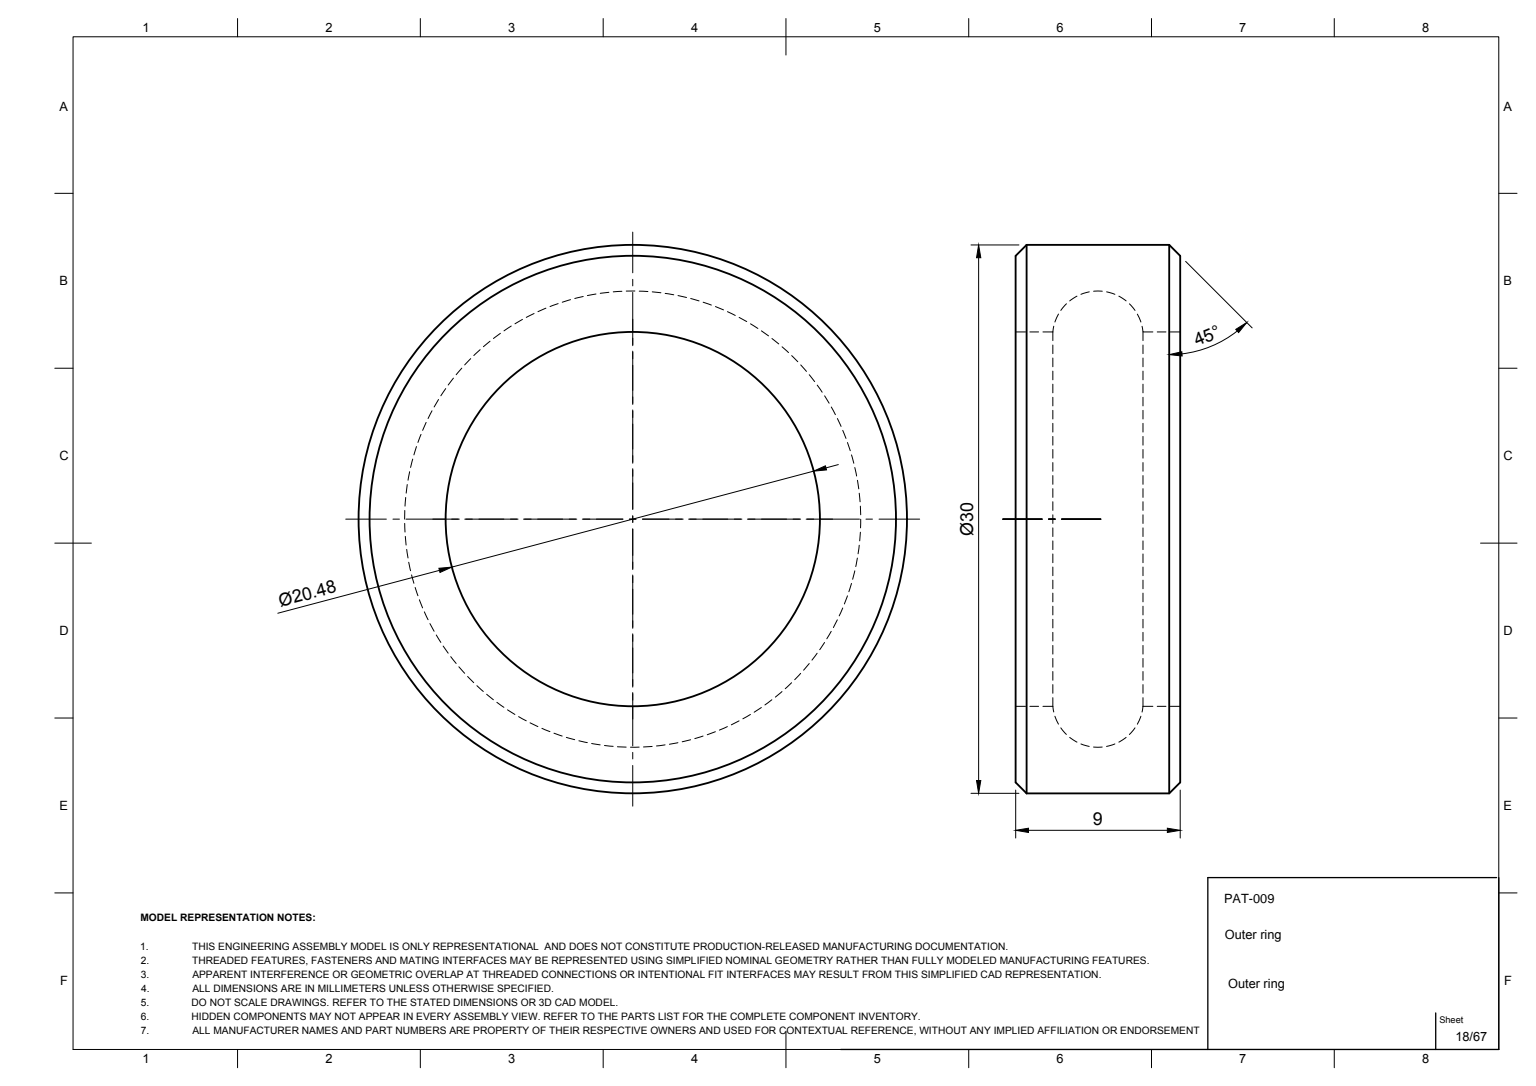
ISO-10303-21;
HEADER;
/* Generated by software containing ST-Developer
 * from STEP Tools, Inc. (www.steptools.com) 
 */

FILE_DESCRIPTION(
/* description */ ('Bell-crank linkage with push rods'),
/* implementation_level */ '2;1');

FILE_NAME(
/* name */ 'Outer ring.step',
/* time_stamp */ '2026-10-28T03:25:15-07:00',
/* author */ (''),
/* organization */ (''),
/* preprocessor_version */ 'ST-DEVELOPER v20.2',
/* originating_system */ 'Autodesk Translation Framework v15.17.0.0',
/* authorisation */ '');

FILE_SCHEMA (('AUTOMOTIVE_DESIGN { 1 0 10303 214 3 1 1 }'));
ENDSEC;

DATA;
#10=MECHANICAL_DESIGN_GEOMETRIC_PRESENTATION_REPRESENTATION('',(#615),#16678);
#432=TOROIDAL_SURFACE('',#9810,1.,0.247676);
#438=CONICAL_SURFACE('',#9821,1.47,0.785398163397449);
#439=CONICAL_SURFACE('',#9825,1.47,0.785398163397449);
#507=SHAPE_REPRESENTATION_RELATIONSHIP('SRR','None',#16924,#561);
#561=ADVANCED_BREP_SHAPE_REPRESENTATION('',(#676),#16629);
#615=STYLED_ITEM('',(#17291),#676);
#676=MANIFOLD_SOLID_BREP('Body1',#8806);
#815=FACE_BOUND('',#2033,.T.);
#816=FACE_BOUND('',#2038,.T.);
#1056=PLANE('',#9818);
#1057=PLANE('',#9827);
#1418=FACE_OUTER_BOUND('',#2030,.T.);
#1419=FACE_OUTER_BOUND('',#2031,.T.);
#1420=FACE_OUTER_BOUND('',#2032,.T.);
#1421=FACE_OUTER_BOUND('',#2034,.T.);
#1422=FACE_OUTER_BOUND('',#2035,.T.);
#1423=FACE_OUTER_BOUND('',#2036,.T.);
#1424=FACE_OUTER_BOUND('',#2037,.T.);
#1425=FACE_OUTER_BOUND('',#2039,.T.);
#2030=EDGE_LOOP('',(#6707,#6708,#6709,#6710,#6711,#6712));
#2031=EDGE_LOOP('',(#6713,#6714,#6715,#6716,#6717));
#2032=EDGE_LOOP('',(#6718));
#2033=EDGE_LOOP('',(#6719));
#2034=EDGE_LOOP('',(#6720,#6721,#6722,#6723));
#2035=EDGE_LOOP('',(#6724,#6725,#6726,#6727));
#2036=EDGE_LOOP('',(#6728,#6729,#6730,#6731));
#2037=EDGE_LOOP('',(#6732));
#2038=EDGE_LOOP('',(#6733));
#2039=EDGE_LOOP('',(#6734,#6735,#6736,#6737,#6738));
#2744=LINE('',#14525,#3293);
#2745=LINE('',#14534,#3294);
#2746=LINE('',#14538,#3295);
#2747=LINE('',#14542,#3296);
#2748=LINE('',#14545,#3297);
#3293=VECTOR('',#11570,1.023815);
#3294=VECTOR('',#11581,1.47);
#3295=VECTOR('',#11586,1.5);
#3296=VECTOR('',#11591,1.47);
#3297=VECTOR('',#11596,1.023815);
#3800=CIRCLE('',#9811,1.023815);
#3801=CIRCLE('',#9812,1.023815);
#3802=CIRCLE('',#9813,0.247676);
#3803=CIRCLE('',#9814,1.023815);
#3804=CIRCLE('',#9815,1.023815);
#3805=CIRCLE('',#9817,1.023815);
#3806=CIRCLE('',#9819,1.44);
#3807=CIRCLE('',#9820,1.023815);
#3808=CIRCLE('',#9822,1.5);
#3809=CIRCLE('',#9824,1.5);
#3810=CIRCLE('',#9826,1.44);
#4373=VERTEX_POINT('',#14513);
#4374=VERTEX_POINT('',#14514);
#4375=VERTEX_POINT('',#14517);
#4376=VERTEX_POINT('',#14519);
#4377=VERTEX_POINT('',#14523);
#4378=VERTEX_POINT('',#14527);
#4379=VERTEX_POINT('',#14529);
#4380=VERTEX_POINT('',#14532);
#4381=VERTEX_POINT('',#14536);
#4382=VERTEX_POINT('',#14540);
#5231=EDGE_CURVE('',#4373,#4374,#3800,.T.);
#5232=EDGE_CURVE('',#4374,#4373,#3801,.T.);
#5233=EDGE_CURVE('',#4374,#4375,#3802,.T.);
#5234=EDGE_CURVE('',#4376,#4375,#3803,.T.);
#5235=EDGE_CURVE('',#4375,#4376,#3804,.T.);
#5236=EDGE_CURVE('',#4377,#4377,#3805,.T.);
#5237=EDGE_CURVE('',#4377,#4376,#2744,.T.);
#5238=EDGE_CURVE('',#4378,#4378,#3806,.T.);
#5239=EDGE_CURVE('',#4379,#4379,#3807,.T.);
#5240=EDGE_CURVE('',#4380,#4380,#3808,.T.);
#5241=EDGE_CURVE('',#4380,#4378,#2745,.T.);
#5242=EDGE_CURVE('',#4381,#4381,#3809,.T.);
#5243=EDGE_CURVE('',#4381,#4380,#2746,.T.);
#5244=EDGE_CURVE('',#4382,#4382,#3810,.T.);
#5245=EDGE_CURVE('',#4382,#4381,#2747,.T.);
#5246=EDGE_CURVE('',#4373,#4379,#2748,.T.);
#6707=ORIENTED_EDGE('',*,*,#5231,.F.);
#6708=ORIENTED_EDGE('',*,*,#5232,.F.);
#6709=ORIENTED_EDGE('',*,*,#5233,.T.);
#6710=ORIENTED_EDGE('',*,*,#5234,.F.);
#6711=ORIENTED_EDGE('',*,*,#5235,.F.);
#6712=ORIENTED_EDGE('',*,*,#5233,.F.);
#6713=ORIENTED_EDGE('',*,*,#5236,.T.);
#6714=ORIENTED_EDGE('',*,*,#5237,.T.);
#6715=ORIENTED_EDGE('',*,*,#5234,.T.);
#6716=ORIENTED_EDGE('',*,*,#5235,.T.);
#6717=ORIENTED_EDGE('',*,*,#5237,.F.);
#6718=ORIENTED_EDGE('',*,*,#5238,.F.);
#6719=ORIENTED_EDGE('',*,*,#5239,.T.);
#6720=ORIENTED_EDGE('',*,*,#5240,.F.);
#6721=ORIENTED_EDGE('',*,*,#5241,.T.);
#6722=ORIENTED_EDGE('',*,*,#5238,.T.);
#6723=ORIENTED_EDGE('',*,*,#5241,.F.);
#6724=ORIENTED_EDGE('',*,*,#5242,.F.);
#6725=ORIENTED_EDGE('',*,*,#5243,.T.);
#6726=ORIENTED_EDGE('',*,*,#5240,.T.);
#6727=ORIENTED_EDGE('',*,*,#5243,.F.);
#6728=ORIENTED_EDGE('',*,*,#5244,.F.);
#6729=ORIENTED_EDGE('',*,*,#5245,.T.);
#6730=ORIENTED_EDGE('',*,*,#5242,.T.);
#6731=ORIENTED_EDGE('',*,*,#5245,.F.);
#6732=ORIENTED_EDGE('',*,*,#5244,.T.);
#6733=ORIENTED_EDGE('',*,*,#5236,.F.);
#6734=ORIENTED_EDGE('',*,*,#5231,.T.);
#6735=ORIENTED_EDGE('',*,*,#5232,.T.);
#6736=ORIENTED_EDGE('',*,*,#5246,.T.);
#6737=ORIENTED_EDGE('',*,*,#5239,.F.);
#6738=ORIENTED_EDGE('',*,*,#5246,.F.);
#8142=CYLINDRICAL_SURFACE('',#9816,1.023815);
#8143=CYLINDRICAL_SURFACE('',#9823,1.5);
#8144=CYLINDRICAL_SURFACE('',#9828,1.023815);
#8443=ADVANCED_FACE('',(#1418),#432,.F.);
#8444=ADVANCED_FACE('',(#1419),#8142,.F.);
#8445=ADVANCED_FACE('',(#1420,#815),#1056,.T.);
#8446=ADVANCED_FACE('',(#1421),#438,.T.);
#8447=ADVANCED_FACE('',(#1422),#8143,.T.);
#8448=ADVANCED_FACE('',(#1423),#439,.T.);
#8449=ADVANCED_FACE('',(#1424,#816),#1057,.T.);
#8450=ADVANCED_FACE('',(#1425),#8144,.F.);
#8806=CLOSED_SHELL('',(#8443,#8444,#8445,#8446,#8447,#8448,#8449,#8450));
#9809=AXIS2_PLACEMENT_3D('',#14511,#11552,#11553);
#9810=AXIS2_PLACEMENT_3D('',#14512,#11554,#11555);
#9811=AXIS2_PLACEMENT_3D('',#14515,#11556,#11557);
#9812=AXIS2_PLACEMENT_3D('',#14516,#11558,#11559);
#9813=AXIS2_PLACEMENT_3D('',#14518,#11560,#11561);
#9814=AXIS2_PLACEMENT_3D('',#14520,#11562,#11563);
#9815=AXIS2_PLACEMENT_3D('',#14521,#11564,#11565);
#9816=AXIS2_PLACEMENT_3D('',#14522,#11566,#11567);
#9817=AXIS2_PLACEMENT_3D('',#14524,#11568,#11569);
#9818=AXIS2_PLACEMENT_3D('',#14526,#11571,#11572);
#9819=AXIS2_PLACEMENT_3D('',#14528,#11573,#11574);
#9820=AXIS2_PLACEMENT_3D('',#14530,#11575,#11576);
#9821=AXIS2_PLACEMENT_3D('',#14531,#11577,#11578);
#9822=AXIS2_PLACEMENT_3D('',#14533,#11579,#11580);
#9823=AXIS2_PLACEMENT_3D('',#14535,#11582,#11583);
#9824=AXIS2_PLACEMENT_3D('',#14537,#11584,#11585);
#9825=AXIS2_PLACEMENT_3D('',#14539,#11587,#11588);
#9826=AXIS2_PLACEMENT_3D('',#14541,#11589,#11590);
#9827=AXIS2_PLACEMENT_3D('',#14543,#11592,#11593);
#9828=AXIS2_PLACEMENT_3D('',#14544,#11594,#11595);
#11552=DIRECTION('axis',(0.,0.,1.));
#11553=DIRECTION('refdir',(1.,0.,0.));
#11554=DIRECTION('center_axis',(0.,-1.,0.));
#11555=DIRECTION('ref_axis',(0.,0.,-1.));
#11556=DIRECTION('center_axis',(0.,-1.,0.));
#11557=DIRECTION('ref_axis',(1.,0.,0.));
#11558=DIRECTION('center_axis',(0.,-1.,0.));
#11559=DIRECTION('ref_axis',(1.,0.,0.));
#11560=DIRECTION('center_axis',(1.,0.,1.22464679914735E-16));
#11561=DIRECTION('ref_axis',(-1.22464679914735E-16,0.,1.));
#11562=DIRECTION('center_axis',(0.,1.,0.));
#11563=DIRECTION('ref_axis',(1.,0.,0.));
#11564=DIRECTION('center_axis',(0.,1.,0.));
#11565=DIRECTION('ref_axis',(1.,0.,0.));
#11566=DIRECTION('center_axis',(0.,-1.,0.));
#11567=DIRECTION('ref_axis',(1.,0.,0.));
#11568=DIRECTION('center_axis',(0.,-1.,0.));
#11569=DIRECTION('ref_axis',(1.,0.,0.));
#11570=DIRECTION('',(0.,1.,0.));
#11571=DIRECTION('center_axis',(0.,1.,0.));
#11572=DIRECTION('ref_axis',(0.,0.,1.));
#11573=DIRECTION('center_axis',(0.,-1.,0.));
#11574=DIRECTION('ref_axis',(1.,0.,0.));
#11575=DIRECTION('center_axis',(0.,-1.,0.));
#11576=DIRECTION('ref_axis',(1.,0.,0.));
#11577=DIRECTION('center_axis',(0.,-1.,0.));
#11578=DIRECTION('ref_axis',(1.,0.,0.));
#11579=DIRECTION('center_axis',(0.,-1.,0.));
#11580=DIRECTION('ref_axis',(1.,0.,0.));
#11581=DIRECTION('',(0.707106781186548,0.707106781186547,8.65956056235494E-17));
#11582=DIRECTION('center_axis',(0.,-1.,0.));
#11583=DIRECTION('ref_axis',(1.,0.,0.));
#11584=DIRECTION('center_axis',(0.,-1.,0.));
#11585=DIRECTION('ref_axis',(1.,0.,0.));
#11586=DIRECTION('',(0.,1.,0.));
#11587=DIRECTION('center_axis',(0.,1.,0.));
#11588=DIRECTION('ref_axis',(1.,0.,0.));
#11589=DIRECTION('center_axis',(0.,-1.,0.));
#11590=DIRECTION('ref_axis',(1.,0.,0.));
#11591=DIRECTION('',(-0.707106781186548,0.707106781186547,-8.65956056235494E-17));
#11592=DIRECTION('center_axis',(0.,-1.,0.));
#11593=DIRECTION('ref_axis',(0.,0.,-1.));
#11594=DIRECTION('center_axis',(0.,-1.,0.));
#11595=DIRECTION('ref_axis',(1.,0.,0.));
#11596=DIRECTION('',(0.,1.,0.));
#14511=CARTESIAN_POINT('',(0.,0.,0.));
#14512=CARTESIAN_POINT('Origin',(0.,0.,0.));
#14513=CARTESIAN_POINT('',(-1.023815,0.246528389340863,-1.25381176266905E-16));
#14514=CARTESIAN_POINT('',(-1.25381176266905E-16,0.246528389340863,1.023815));
#14515=CARTESIAN_POINT('Origin',(0.,0.246528389340863,0.));
#14516=CARTESIAN_POINT('Origin',(0.,0.246528389340863,0.));
#14517=CARTESIAN_POINT('',(-1.25381176266905E-16,-0.246528389340863,1.023815));
#14518=CARTESIAN_POINT('Origin',(-1.22464679914735E-16,0.,1.));
#14519=CARTESIAN_POINT('',(-1.023815,-0.246528389340863,1.25381176266905E-16));
#14520=CARTESIAN_POINT('Origin',(0.,-0.246528389340863,0.));
#14521=CARTESIAN_POINT('Origin',(0.,-0.246528389340863,0.));
#14522=CARTESIAN_POINT('Origin',(0.,0.,0.));
#14523=CARTESIAN_POINT('',(-1.023815,-0.45,-1.25381176266905E-16));
#14524=CARTESIAN_POINT('Origin',(0.,-0.45,0.));
#14525=CARTESIAN_POINT('',(-1.023815,0.,-1.25381176266905E-16));
#14526=CARTESIAN_POINT('Origin',(1.44,0.45,0.));
#14527=CARTESIAN_POINT('',(-1.44,0.45,-1.76349139077219E-16));
#14528=CARTESIAN_POINT('Origin',(0.,0.45,0.));
#14529=CARTESIAN_POINT('',(-1.023815,0.45,-1.25381176266905E-16));
#14530=CARTESIAN_POINT('Origin',(0.,0.45,0.));
#14531=CARTESIAN_POINT('Origin',(0.,0.42,0.));
#14532=CARTESIAN_POINT('',(-1.5,0.39,-1.83697019872103E-16));
#14533=CARTESIAN_POINT('Origin',(0.,0.39,0.));
#14534=CARTESIAN_POINT('',(-1.47,0.42,-1.80023079474661E-16));
#14535=CARTESIAN_POINT('Origin',(0.,0.,0.));
#14536=CARTESIAN_POINT('',(-1.5,-0.39,-1.83697019872103E-16));
#14537=CARTESIAN_POINT('Origin',(0.,-0.39,0.));
#14538=CARTESIAN_POINT('',(-1.5,0.,-1.83697019872103E-16));
#14539=CARTESIAN_POINT('Origin',(0.,-0.42,0.));
#14540=CARTESIAN_POINT('',(-1.44,-0.45,-1.76349139077219E-16));
#14541=CARTESIAN_POINT('Origin',(0.,-0.45,0.));
#14542=CARTESIAN_POINT('',(-1.47,-0.42,-1.80023079474661E-16));
#14543=CARTESIAN_POINT('Origin',(1.023815,-0.45,0.));
#14544=CARTESIAN_POINT('Origin',(0.,0.,0.));
#14545=CARTESIAN_POINT('',(-1.023815,0.,-1.25381176266905E-16));
#16565=UNCERTAINTY_MEASURE_WITH_UNIT(LENGTH_MEASURE(0.001),#16679,
'DISTANCE_ACCURACY_VALUE',
'Maximum model space distance between geometric entities at asserted c
onnectivities');
#16614=UNCERTAINTY_MEASURE_WITH_UNIT(LENGTH_MEASURE(0.001),#16679,
'DISTANCE_ACCURACY_VALUE',
'Maximum model space distance between geometric entities at asserted c
onnectivities');
#16629=(
GEOMETRIC_REPRESENTATION_CONTEXT(3)
GLOBAL_UNCERTAINTY_ASSIGNED_CONTEXT((#16565))
GLOBAL_UNIT_ASSIGNED_CONTEXT((#16679,#16681,#16682))
REPRESENTATION_CONTEXT('','3D')
);
#16678=(
GEOMETRIC_REPRESENTATION_CONTEXT(3)
GLOBAL_UNCERTAINTY_ASSIGNED_CONTEXT((#16614))
GLOBAL_UNIT_ASSIGNED_CONTEXT((#16679,#16681,#16682))
REPRESENTATION_CONTEXT('','3D')
);
#16679=(
LENGTH_UNIT()
NAMED_UNIT(*)
SI_UNIT(.CENTI.,.METRE.)
);
#16681=(
NAMED_UNIT(*)
PLANE_ANGLE_UNIT()
SI_UNIT($,.RADIAN.)
);
#16682=(
NAMED_UNIT(*)
SI_UNIT($,.STERADIAN.)
SOLID_ANGLE_UNIT()
);
#16697=SHAPE_DEFINITION_REPRESENTATION(#16760,#16924);
#16760=PRODUCT_DEFINITION_SHAPE('',$,#16988);
#16924=SHAPE_REPRESENTATION('',(#9809),#16629);
#16973=PRODUCT_DEFINITION_CONTEXT('part definition',#17164,'design');
#16988=PRODUCT_DEFINITION('Outer ring','Outer ring',#17051,#16973);
#17051=PRODUCT_DEFINITION_FORMATION('',$,#17180);
#17164=APPLICATION_CONTEXT(
'Core Data for Automotive Mechanical Design Process');
#17165=PRODUCT_CONTEXT('part definition',#17164,'mechanical');
#17180=PRODUCT('Outer ring','Outer ring','Outer ring',(#17165));
#17285=COLOUR_RGB('Grey',0.48,0.52,0.57);
#17286=FILL_AREA_STYLE_COLOUR('',#17285);
#17287=FILL_AREA_STYLE('',(#17286));
#17288=SURFACE_STYLE_FILL_AREA(#17287);
#17289=SURFACE_SIDE_STYLE('',(#17288));
#17290=SURFACE_STYLE_USAGE(.BOTH.,#17289);
#17291=PRESENTATION_STYLE_ASSIGNMENT((#17290));
ENDSEC;
END-ISO-10303-21;
